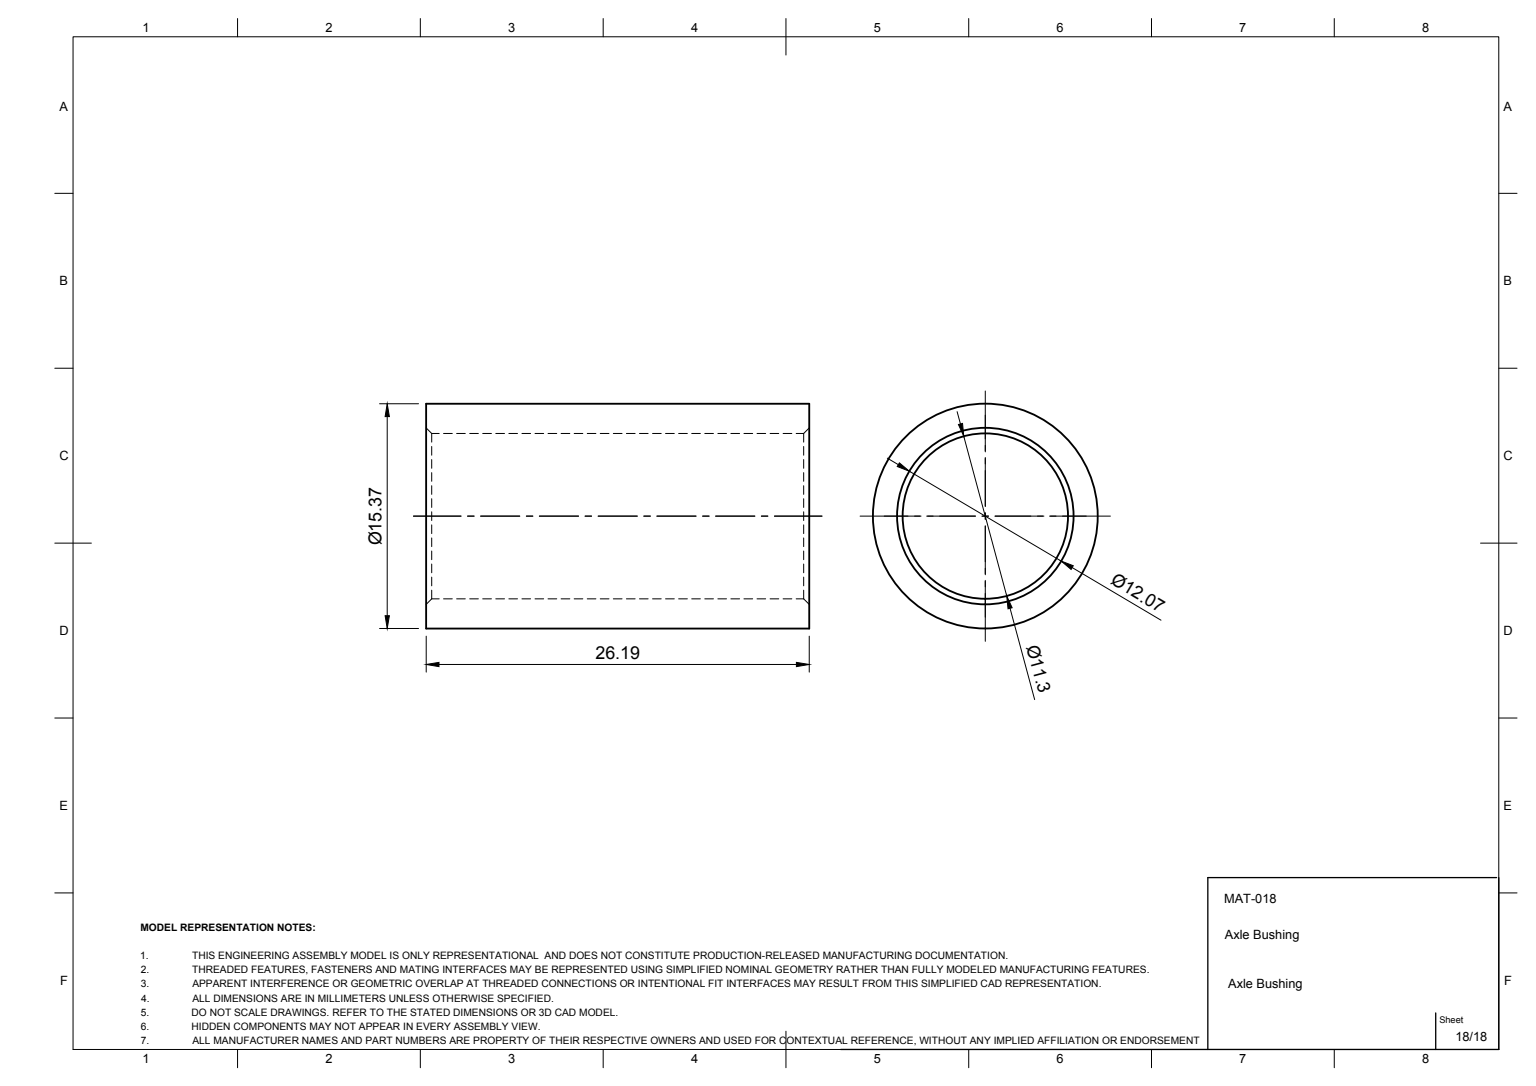
ISO-10303-21;
HEADER;
/* Generated by software containing ST-Developer
 * from STEP Tools, Inc. (www.steptools.com) 
 */

FILE_DESCRIPTION(
/* description */ ('STEP AP214'),
/* implementation_level */ '2;1');

FILE_NAME(
/* name */ 'Axle Bushing.step',
/* time_stamp */ '2026-11-14T06:16:09-08:00',
/* author */ (''),
/* organization */ (''),
/* preprocessor_version */ 'ST-DEVELOPER v20.2',
/* originating_system */ 'Autodesk Translation Framework v15.17.0.0',
/* authorisation */ '');

FILE_SCHEMA (('AUTOMOTIVE_DESIGN { 1 0 10303 214 3 1 1 }'));
ENDSEC;

DATA;
#10=MECHANICAL_DESIGN_GEOMETRIC_PRESENTATION_REPRESENTATION('',(#362),#18006);
#151=CONICAL_SURFACE('',#10827,6.0325,0.785398163397448);
#152=CONICAL_SURFACE('',#10833,5.6515,0.785398163397444);
#330=SHAPE_REPRESENTATION_RELATIONSHIP('SRR','None',#18088,#346);
#346=ADVANCED_BREP_SHAPE_REPRESENTATION('',(#378),#18005);
#362=STYLED_ITEM('',(#18171),#378);
#378=MANIFOLD_SOLID_BREP('Body1',#9571);
#500=FACE_BOUND('',#2113,.T.);
#501=FACE_BOUND('',#2115,.T.);
#839=PLANE('',#10838);
#840=PLANE('',#10839);
#1411=FACE_OUTER_BOUND('',#2108,.T.);
#1412=FACE_OUTER_BOUND('',#2109,.T.);
#1413=FACE_OUTER_BOUND('',#2110,.T.);
#1414=FACE_OUTER_BOUND('',#2111,.T.);
#1415=FACE_OUTER_BOUND('',#2112,.T.);
#1416=FACE_OUTER_BOUND('',#2114,.T.);
#2108=EDGE_LOOP('',(#8786,#8787,#8788,#8789,#8790));
#2109=EDGE_LOOP('',(#8791,#8792,#8793,#8794,#8795));
#2110=EDGE_LOOP('',(#8796,#8797,#8798,#8799));
#2111=EDGE_LOOP('',(#8800,#8801,#8802,#8803));
#2112=EDGE_LOOP('',(#8804));
#2113=EDGE_LOOP('',(#8805));
#2114=EDGE_LOOP('',(#8806));
#2115=EDGE_LOOP('',(#8807));
#2836=LINE('',#17927,#3560);
#2837=LINE('',#17932,#3561);
#2838=LINE('',#17936,#3562);
#2839=LINE('',#17942,#3563);
#3560=VECTOR('',#13741,6.0325);
#3561=VECTOR('',#13748,5.6515);
#3562=VECTOR('',#13753,5.6515);
#3563=VECTOR('',#13760,7.6835);
#4006=CIRCLE('',#10828,5.6515);
#4007=CIRCLE('',#10829,6.0325);
#4008=CIRCLE('',#10830,5.6515);
#4009=CIRCLE('',#10832,5.6515);
#4010=CIRCLE('',#10834,6.0325);
#4011=CIRCLE('',#10836,7.6835);
#4012=CIRCLE('',#10837,7.6835);
#4817=VERTEX_POINT('',#17923);
#4818=VERTEX_POINT('',#17924);
#4819=VERTEX_POINT('',#17926);
#4820=VERTEX_POINT('',#17931);
#4821=VERTEX_POINT('',#17935);
#4822=VERTEX_POINT('',#17939);
#4823=VERTEX_POINT('',#17941);
#6141=EDGE_CURVE('',#4817,#4818,#4006,.T.);
#6142=EDGE_CURVE('',#4818,#4819,#2836,.T.);
#6143=EDGE_CURVE('',#4819,#4819,#4007,.T.);
#6144=EDGE_CURVE('',#4818,#4817,#4008,.T.);
#6145=EDGE_CURVE('',#4817,#4820,#2837,.T.);
#6146=EDGE_CURVE('',#4820,#4820,#4009,.T.);
#6147=EDGE_CURVE('',#4820,#4821,#2838,.T.);
#6148=EDGE_CURVE('',#4821,#4821,#4010,.T.);
#6149=EDGE_CURVE('',#4822,#4822,#4011,.T.);
#6150=EDGE_CURVE('',#4822,#4823,#2839,.T.);
#6151=EDGE_CURVE('',#4823,#4823,#4012,.T.);
#8786=ORIENTED_EDGE('',*,*,#6141,.T.);
#8787=ORIENTED_EDGE('',*,*,#6142,.T.);
#8788=ORIENTED_EDGE('',*,*,#6143,.F.);
#8789=ORIENTED_EDGE('',*,*,#6142,.F.);
#8790=ORIENTED_EDGE('',*,*,#6144,.T.);
#8791=ORIENTED_EDGE('',*,*,#6141,.F.);
#8792=ORIENTED_EDGE('',*,*,#6145,.T.);
#8793=ORIENTED_EDGE('',*,*,#6146,.T.);
#8794=ORIENTED_EDGE('',*,*,#6145,.F.);
#8795=ORIENTED_EDGE('',*,*,#6144,.F.);
#8796=ORIENTED_EDGE('',*,*,#6146,.F.);
#8797=ORIENTED_EDGE('',*,*,#6147,.T.);
#8798=ORIENTED_EDGE('',*,*,#6148,.T.);
#8799=ORIENTED_EDGE('',*,*,#6147,.F.);
#8800=ORIENTED_EDGE('',*,*,#6149,.F.);
#8801=ORIENTED_EDGE('',*,*,#6150,.T.);
#8802=ORIENTED_EDGE('',*,*,#6151,.T.);
#8803=ORIENTED_EDGE('',*,*,#6150,.F.);
#8804=ORIENTED_EDGE('',*,*,#6149,.T.);
#8805=ORIENTED_EDGE('',*,*,#6148,.F.);
#8806=ORIENTED_EDGE('',*,*,#6151,.F.);
#8807=ORIENTED_EDGE('',*,*,#6143,.T.);
#8978=CYLINDRICAL_SURFACE('',#10831,5.6515);
#8979=CYLINDRICAL_SURFACE('',#10835,7.6835);
#9550=ADVANCED_FACE('',(#1411),#151,.F.);
#9551=ADVANCED_FACE('',(#1412),#8978,.F.);
#9552=ADVANCED_FACE('',(#1413),#152,.F.);
#9553=ADVANCED_FACE('',(#1414),#8979,.T.);
#9554=ADVANCED_FACE('',(#1415,#500),#839,.T.);
#9555=ADVANCED_FACE('',(#1416,#501),#840,.T.);
#9571=CLOSED_SHELL('',(#9550,#9551,#9552,#9553,#9554,#9555));
#10826=AXIS2_PLACEMENT_3D('',#17921,#13735,#13736);
#10827=AXIS2_PLACEMENT_3D('',#17922,#13737,#13738);
#10828=AXIS2_PLACEMENT_3D('',#17925,#13739,#13740);
#10829=AXIS2_PLACEMENT_3D('',#17928,#13742,#13743);
#10830=AXIS2_PLACEMENT_3D('',#17929,#13744,#13745);
#10831=AXIS2_PLACEMENT_3D('',#17930,#13746,#13747);
#10832=AXIS2_PLACEMENT_3D('',#17933,#13749,#13750);
#10833=AXIS2_PLACEMENT_3D('',#17934,#13751,#13752);
#10834=AXIS2_PLACEMENT_3D('',#17937,#13754,#13755);
#10835=AXIS2_PLACEMENT_3D('',#17938,#13756,#13757);
#10836=AXIS2_PLACEMENT_3D('',#17940,#13758,#13759);
#10837=AXIS2_PLACEMENT_3D('',#17943,#13761,#13762);
#10838=AXIS2_PLACEMENT_3D('',#17944,#13763,#13764);
#10839=AXIS2_PLACEMENT_3D('',#17945,#13765,#13766);
#13735=DIRECTION('axis',(0.,0.,1.));
#13736=DIRECTION('refdir',(1.,0.,0.));
#13737=DIRECTION('center_axis',(0.,0.,1.));
#13738=DIRECTION('ref_axis',(1.,0.,0.));
#13739=DIRECTION('center_axis',(0.,0.,-1.));
#13740=DIRECTION('ref_axis',(-1.,0.,0.));
#13741=DIRECTION('',(-0.707106781186547,-8.65956056235493E-17,0.707106781186548));
#13742=DIRECTION('center_axis',(0.,0.,-1.));
#13743=DIRECTION('ref_axis',(-1.,0.,0.));
#13744=DIRECTION('center_axis',(0.,0.,-1.));
#13745=DIRECTION('ref_axis',(-1.,0.,0.));
#13746=DIRECTION('center_axis',(0.,0.,-1.));
#13747=DIRECTION('ref_axis',(-1.,0.,0.));
#13748=DIRECTION('',(0.,0.,-1.));
#13749=DIRECTION('center_axis',(0.,0.,-1.));
#13750=DIRECTION('ref_axis',(-1.,0.,0.));
#13751=DIRECTION('center_axis',(0.,0.,-1.));
#13752=DIRECTION('ref_axis',(-1.,0.,0.));
#13753=DIRECTION('',(0.707106781186545,-8.6595605623549E-17,-0.707106781186551));
#13754=DIRECTION('center_axis',(0.,0.,-1.));
#13755=DIRECTION('ref_axis',(-1.,0.,0.));
#13756=DIRECTION('center_axis',(0.,0.,-1.));
#13757=DIRECTION('ref_axis',(-1.,0.,0.));
#13758=DIRECTION('center_axis',(0.,0.,-1.));
#13759=DIRECTION('ref_axis',(-1.,0.,0.));
#13760=DIRECTION('',(0.,0.,1.));
#13761=DIRECTION('center_axis',(0.,0.,-1.));
#13762=DIRECTION('ref_axis',(-1.,0.,0.));
#13763=DIRECTION('center_axis',(0.,0.,-1.));
#13764=DIRECTION('ref_axis',(0.,-1.,0.));
#13765=DIRECTION('center_axis',(0.,0.,1.));
#13766=DIRECTION('ref_axis',(1.,0.,0.));
#17921=CARTESIAN_POINT('',(0.,0.,0.));
#17922=CARTESIAN_POINT('Origin',(0.,0.,13.09624));
#17923=CARTESIAN_POINT('',(5.6515,6.92109138538127E-16,12.71524));
#17924=CARTESIAN_POINT('',(-5.6515,-6.92109138538127E-16,12.71524));
#17925=CARTESIAN_POINT('Origin',(0.,0.,12.71524));
#17926=CARTESIAN_POINT('',(-6.0325,-7.38768181585641E-16,13.09624));
#17927=CARTESIAN_POINT('',(-6.0325,-7.38768181585641E-16,13.09624));
#17928=CARTESIAN_POINT('Origin',(0.,0.,13.09624));
#17929=CARTESIAN_POINT('Origin',(0.,0.,12.71524));
#17930=CARTESIAN_POINT('Origin',(0.,0.,-13.09624));
#17931=CARTESIAN_POINT('',(5.6515,-6.92109138538127E-16,-12.71524));
#17932=CARTESIAN_POINT('',(5.6515,-6.92109138538127E-16,-13.09624));
#17933=CARTESIAN_POINT('Origin',(0.,0.,-12.71524));
#17934=CARTESIAN_POINT('Origin',(0.,0.,-12.71524));
#17935=CARTESIAN_POINT('',(6.0325,-7.38768181585641E-16,-13.09624));
#17936=CARTESIAN_POINT('',(5.6515,-6.92109138538127E-16,-12.71524));
#17937=CARTESIAN_POINT('Origin',(0.,0.,-13.09624));
#17938=CARTESIAN_POINT('Origin',(0.,0.,-13.09624));
#17939=CARTESIAN_POINT('',(7.6835,-9.40957368124869E-16,-13.09624));
#17940=CARTESIAN_POINT('Origin',(0.,0.,-13.09624));
#17941=CARTESIAN_POINT('',(7.6835,-9.40957368124869E-16,13.09624));
#17942=CARTESIAN_POINT('',(7.6835,-9.40957368124869E-16,-13.09624));
#17943=CARTESIAN_POINT('Origin',(0.,0.,13.09624));
#17944=CARTESIAN_POINT('Origin',(0.,6.0325,-13.09624));
#17945=CARTESIAN_POINT('Origin',(0.,7.6835,13.09624));
#17985=UNCERTAINTY_MEASURE_WITH_UNIT(LENGTH_MEASURE(0.01),#18007,
'DISTANCE_ACCURACY_VALUE',
'Maximum model space distance between geometric entities at asserted c
onnectivities');
#17986=UNCERTAINTY_MEASURE_WITH_UNIT(LENGTH_MEASURE(0.01),#18007,
'DISTANCE_ACCURACY_VALUE',
'Maximum model space distance between geometric entities at asserted c
onnectivities');
#18005=(
GEOMETRIC_REPRESENTATION_CONTEXT(3)
GLOBAL_UNCERTAINTY_ASSIGNED_CONTEXT((#17985))
GLOBAL_UNIT_ASSIGNED_CONTEXT((#18007,#18009,#18010))
REPRESENTATION_CONTEXT('','3D')
);
#18006=(
GEOMETRIC_REPRESENTATION_CONTEXT(3)
GLOBAL_UNCERTAINTY_ASSIGNED_CONTEXT((#17986))
GLOBAL_UNIT_ASSIGNED_CONTEXT((#18007,#18009,#18010))
REPRESENTATION_CONTEXT('','3D')
);
#18007=(
LENGTH_UNIT()
NAMED_UNIT(*)
SI_UNIT(.MILLI.,.METRE.)
);
#18009=(
NAMED_UNIT(*)
PLANE_ANGLE_UNIT()
SI_UNIT($,.RADIAN.)
);
#18010=(
NAMED_UNIT(*)
SI_UNIT($,.STERADIAN.)
SOLID_ANGLE_UNIT()
);
#18029=SHAPE_DEFINITION_REPRESENTATION(#18048,#18088);
#18048=PRODUCT_DEFINITION_SHAPE('',$,#18108);
#18088=SHAPE_REPRESENTATION('',(#10826),#18005);
#18089=PRODUCT_DEFINITION_CONTEXT('part definition',#18148,'design');
#18108=PRODUCT_DEFINITION('Axle Bushing','Axle Bushing',#18127,#18089);
#18127=PRODUCT_DEFINITION_FORMATION('',$,#18168);
#18148=APPLICATION_CONTEXT(
'Core Data for Automotive Mechanical Design Process');
#18149=PRODUCT_CONTEXT('part definition',#18148,'mechanical');
#18168=PRODUCT('Axle Bushing','Axle Bushing',$,(#18149));
#18171=PRESENTATION_STYLE_ASSIGNMENT((#18175));
#18175=SURFACE_STYLE_USAGE(.BOTH.,#18179);
#18179=SURFACE_SIDE_STYLE('',(#18183));
#18183=SURFACE_STYLE_FILL_AREA(#18187);
#18187=FILL_AREA_STYLE('Opaque(61,176,222)',(#18191));
#18191=FILL_AREA_STYLE_COLOUR('Opaque(61,176,222)',#18195);
#18195=COLOUR_RGB('Opaque(61,176,222)',0.23921568627451,0.690196078431373,
0.870588235294118);
ENDSEC;
END-ISO-10303-21;
